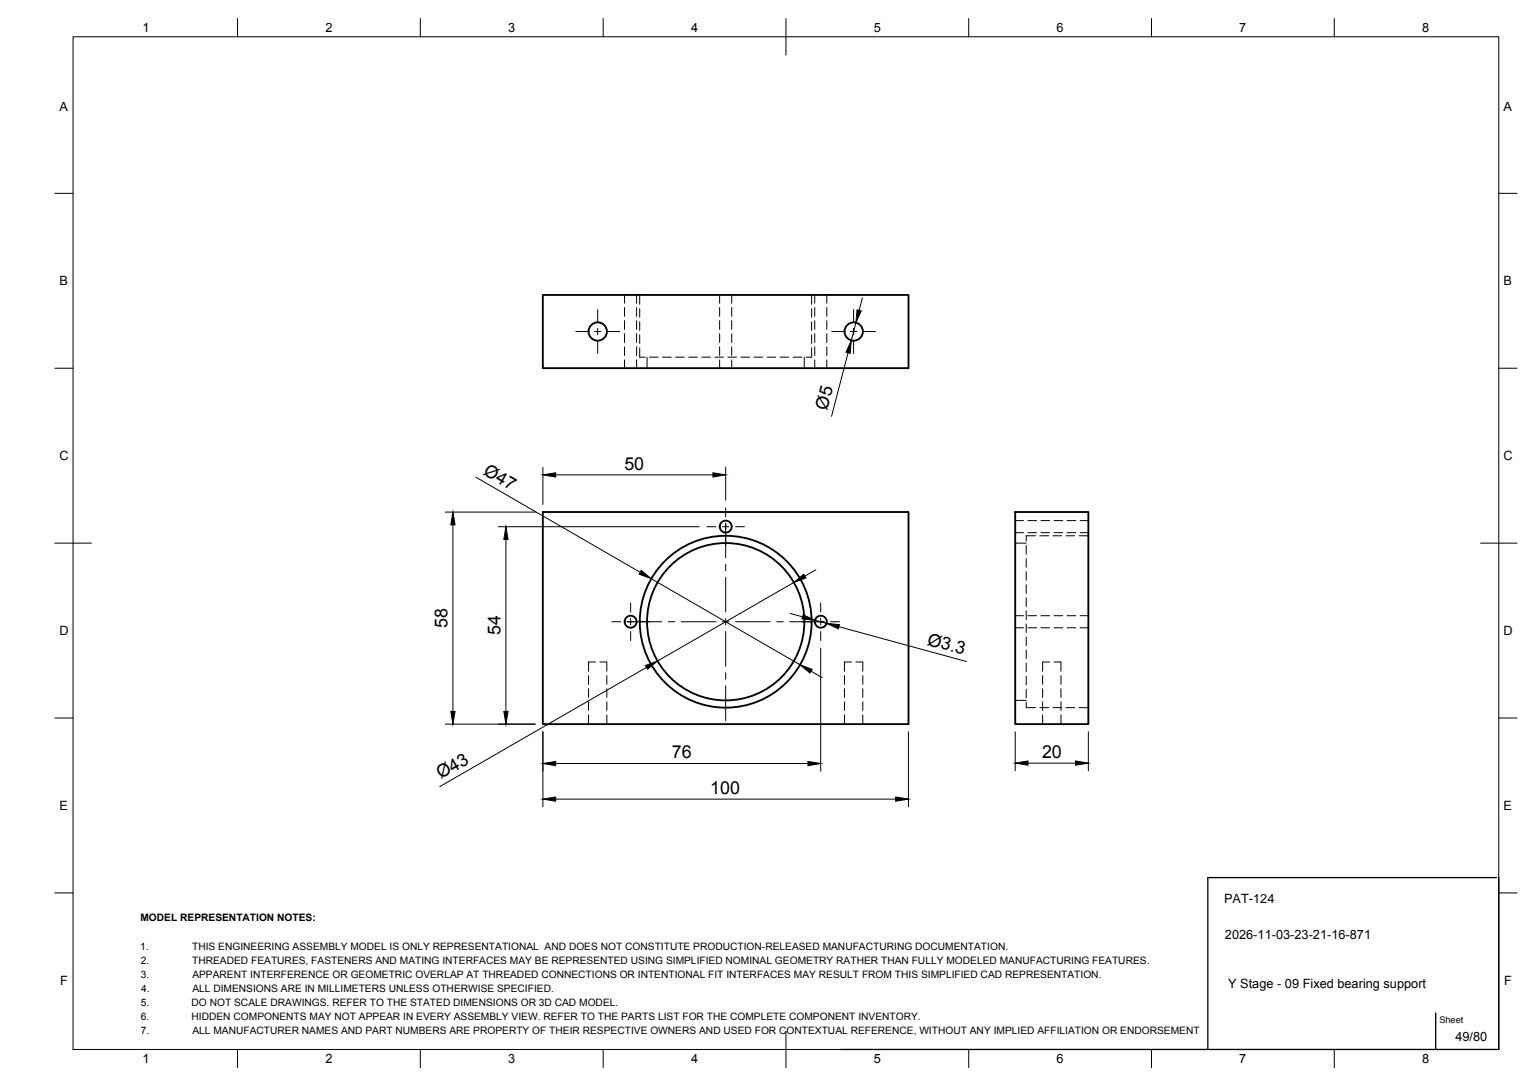
ISO-10303-21;
HEADER;
/* Generated by software containing ST-Developer
 * from STEP Tools, Inc. (www.steptools.com) 
 */

FILE_DESCRIPTION(
/* description */ ('XY cross-slide table'),
/* implementation_level */ '2;1');

FILE_NAME(
/* name */ 'Y Stage - 09 Fixed bearing support.step',
/* time_stamp */ '2026-10-28T03:22:46-07:00',
/* author */ (''),
/* organization */ (''),
/* preprocessor_version */ 'ST-DEVELOPER v20.2',
/* originating_system */ 'Autodesk Translation Framework v15.17.0.0',
/* authorisation */ '');

FILE_SCHEMA (('AUTOMOTIVE_DESIGN { 1 0 10303 214 3 1 1 }'));
ENDSEC;

DATA;
#10=MECHANICAL_DESIGN_GEOMETRIC_PRESENTATION_REPRESENTATION('',(#1731),#62984);
#1550=SHAPE_REPRESENTATION_RELATIONSHIP('SRR','None',#63405,#1633);
#1633=ADVANCED_BREP_SHAPE_REPRESENTATION('',(#1840),#62942);
#1731=STYLED_ITEM('',(#63912),#1840);
#1840=MANIFOLD_SOLID_BREP('Body1',#23029);
#2163=FACE_BOUND('',#5200,.T.);
#2164=FACE_BOUND('',#5208,.T.);
#2165=FACE_BOUND('',#5209,.T.);
#2166=FACE_BOUND('',#5210,.T.);
#2167=FACE_BOUND('',#5211,.T.);
#2168=FACE_BOUND('',#5214,.T.);
#2169=FACE_BOUND('',#5215,.T.);
#2170=FACE_BOUND('',#5216,.T.);
#2171=FACE_BOUND('',#5217,.T.);
#2172=FACE_BOUND('',#5220,.T.);
#2173=FACE_BOUND('',#5221,.T.);
#2617=PLANE('',#25418);
#2618=PLANE('',#25425);
#2619=PLANE('',#25429);
#2620=PLANE('',#25430);
#2621=PLANE('',#25431);
#2622=PLANE('',#25432);
#2623=PLANE('',#25433);
#2624=PLANE('',#25434);
#2625=PLANE('',#25435);
#3605=FACE_OUTER_BOUND('',#5195,.T.);
#3606=FACE_OUTER_BOUND('',#5196,.T.);
#3607=FACE_OUTER_BOUND('',#5197,.T.);
#3608=FACE_OUTER_BOUND('',#5198,.T.);
#3609=FACE_OUTER_BOUND('',#5199,.T.);
#3610=FACE_OUTER_BOUND('',#5201,.T.);
#3611=FACE_OUTER_BOUND('',#5202,.T.);
#3612=FACE_OUTER_BOUND('',#5203,.T.);
#3613=FACE_OUTER_BOUND('',#5204,.T.);
#3614=FACE_OUTER_BOUND('',#5205,.T.);
#3615=FACE_OUTER_BOUND('',#5206,.T.);
#3616=FACE_OUTER_BOUND('',#5207,.T.);
#3617=FACE_OUTER_BOUND('',#5212,.T.);
#3618=FACE_OUTER_BOUND('',#5213,.T.);
#3619=FACE_OUTER_BOUND('',#5218,.T.);
#3620=FACE_OUTER_BOUND('',#5219,.T.);
#5195=EDGE_LOOP('',(#18328,#18329,#18330,#18331));
#5196=EDGE_LOOP('',(#18332,#18333,#18334,#18335));
#5197=EDGE_LOOP('',(#18336,#18337,#18338,#18339));
#5198=EDGE_LOOP('',(#18340,#18341,#18342,#18343));
#5199=EDGE_LOOP('',(#18344));
#5200=EDGE_LOOP('',(#18345));
#5201=EDGE_LOOP('',(#18346,#18347,#18348,#18349));
#5202=EDGE_LOOP('',(#18350,#18351,#18352,#18353));
#5203=EDGE_LOOP('',(#18354));
#5204=EDGE_LOOP('',(#18355,#18356,#18357,#18358));
#5205=EDGE_LOOP('',(#18359));
#5206=EDGE_LOOP('',(#18360,#18361,#18362,#18363));
#5207=EDGE_LOOP('',(#18364,#18365,#18366,#18367));
#5208=EDGE_LOOP('',(#18368));
#5209=EDGE_LOOP('',(#18369));
#5210=EDGE_LOOP('',(#18370));
#5211=EDGE_LOOP('',(#18371));
#5212=EDGE_LOOP('',(#18372,#18373,#18374,#18375));
#5213=EDGE_LOOP('',(#18376,#18377,#18378,#18379));
#5214=EDGE_LOOP('',(#18380));
#5215=EDGE_LOOP('',(#18381));
#5216=EDGE_LOOP('',(#18382));
#5217=EDGE_LOOP('',(#18383));
#5218=EDGE_LOOP('',(#18384,#18385,#18386,#18387));
#5219=EDGE_LOOP('',(#18388,#18389,#18390,#18391));
#5220=EDGE_LOOP('',(#18392));
#5221=EDGE_LOOP('',(#18393));
#6737=LINE('',#48212,#8224);
#6738=LINE('',#48218,#8225);
#6739=LINE('',#48224,#8226);
#6740=LINE('',#48230,#8227);
#6741=LINE('',#48238,#8228);
#6742=LINE('',#48243,#8229);
#6743=LINE('',#48250,#8230);
#6744=LINE('',#48256,#8231);
#6745=LINE('',#48258,#8232);
#6746=LINE('',#48260,#8233);
#6747=LINE('',#48261,#8234);
#6748=LINE('',#48264,#8235);
#6749=LINE('',#48266,#8236);
#6750=LINE('',#48267,#8237);
#6751=LINE('',#48270,#8238);
#6752=LINE('',#48272,#8239);
#6753=LINE('',#48273,#8240);
#6754=LINE('',#48275,#8241);
#6755=LINE('',#48276,#8242);
#8224=VECTOR('',#30108,0.165);
#8225=VECTOR('',#30115,0.165);
#8226=VECTOR('',#30122,0.165);
#8227=VECTOR('',#30129,2.35);
#8228=VECTOR('',#30140,2.15);
#8229=VECTOR('',#30145,0.25);
#8230=VECTOR('',#30154,0.25);
#8231=VECTOR('',#30161,1.);
#8232=VECTOR('',#30162,1.);
#8233=VECTOR('',#30163,1.);
#8234=VECTOR('',#30164,1.);
#8235=VECTOR('',#30167,1.);
#8236=VECTOR('',#30168,1.);
#8237=VECTOR('',#30169,1.);
#8238=VECTOR('',#30172,1.);
#8239=VECTOR('',#30173,1.);
#8240=VECTOR('',#30174,1.);
#8241=VECTOR('',#30177,1.);
#8242=VECTOR('',#30178,1.);
#9417=CIRCLE('',#25407,0.165);
#9418=CIRCLE('',#25408,0.165);
#9419=CIRCLE('',#25410,0.165);
#9420=CIRCLE('',#25411,0.165);
#9421=CIRCLE('',#25413,0.165);
#9422=CIRCLE('',#25414,0.165);
#9423=CIRCLE('',#25416,2.35);
#9424=CIRCLE('',#25417,2.35);
#9425=CIRCLE('',#25419,2.15);
#9426=CIRCLE('',#25421,2.15);
#9427=CIRCLE('',#25423,0.25);
#9428=CIRCLE('',#25424,0.25);
#9429=CIRCLE('',#25427,0.25);
#9430=CIRCLE('',#25428,0.25);
#10921=VERTEX_POINT('',#48209);
#10922=VERTEX_POINT('',#48211);
#10923=VERTEX_POINT('',#48215);
#10924=VERTEX_POINT('',#48217);
#10925=VERTEX_POINT('',#48221);
#10926=VERTEX_POINT('',#48223);
#10927=VERTEX_POINT('',#48227);
#10928=VERTEX_POINT('',#48229);
#10929=VERTEX_POINT('',#48233);
#10930=VERTEX_POINT('',#48236);
#10931=VERTEX_POINT('',#48240);
#10932=VERTEX_POINT('',#48242);
#10933=VERTEX_POINT('',#48247);
#10934=VERTEX_POINT('',#48249);
#10935=VERTEX_POINT('',#48254);
#10936=VERTEX_POINT('',#48255);
#10937=VERTEX_POINT('',#48257);
#10938=VERTEX_POINT('',#48259);
#10939=VERTEX_POINT('',#48263);
#10940=VERTEX_POINT('',#48265);
#10941=VERTEX_POINT('',#48269);
#10942=VERTEX_POINT('',#48271);
#13548=EDGE_CURVE('',#10921,#10921,#9417,.T.);
#13549=EDGE_CURVE('',#10921,#10922,#6737,.T.);
#13550=EDGE_CURVE('',#10922,#10922,#9418,.T.);
#13551=EDGE_CURVE('',#10923,#10923,#9419,.T.);
#13552=EDGE_CURVE('',#10923,#10924,#6738,.T.);
#13553=EDGE_CURVE('',#10924,#10924,#9420,.T.);
#13554=EDGE_CURVE('',#10925,#10925,#9421,.T.);
#13555=EDGE_CURVE('',#10925,#10926,#6739,.T.);
#13556=EDGE_CURVE('',#10926,#10926,#9422,.T.);
#13557=EDGE_CURVE('',#10927,#10927,#9423,.T.);
#13558=EDGE_CURVE('',#10927,#10928,#6740,.T.);
#13559=EDGE_CURVE('',#10928,#10928,#9424,.T.);
#13560=EDGE_CURVE('',#10929,#10929,#9425,.T.);
#13561=EDGE_CURVE('',#10930,#10930,#9426,.T.);
#13562=EDGE_CURVE('',#10930,#10929,#6741,.T.);
#13563=EDGE_CURVE('',#10931,#10931,#9427,.T.);
#13564=EDGE_CURVE('',#10931,#10932,#6742,.T.);
#13565=EDGE_CURVE('',#10932,#10932,#9428,.T.);
#13566=EDGE_CURVE('',#10933,#10933,#9429,.T.);
#13567=EDGE_CURVE('',#10933,#10934,#6743,.T.);
#13568=EDGE_CURVE('',#10934,#10934,#9430,.T.);
#13569=EDGE_CURVE('',#10935,#10936,#6744,.T.);
#13570=EDGE_CURVE('',#10936,#10937,#6745,.T.);
#13571=EDGE_CURVE('',#10938,#10937,#6746,.T.);
#13572=EDGE_CURVE('',#10935,#10938,#6747,.T.);
#13573=EDGE_CURVE('',#10939,#10935,#6748,.T.);
#13574=EDGE_CURVE('',#10940,#10938,#6749,.T.);
#13575=EDGE_CURVE('',#10939,#10940,#6750,.T.);
#13576=EDGE_CURVE('',#10941,#10939,#6751,.T.);
#13577=EDGE_CURVE('',#10942,#10940,#6752,.T.);
#13578=EDGE_CURVE('',#10941,#10942,#6753,.T.);
#13579=EDGE_CURVE('',#10936,#10941,#6754,.T.);
#13580=EDGE_CURVE('',#10937,#10942,#6755,.T.);
#18328=ORIENTED_EDGE('',*,*,#13548,.F.);
#18329=ORIENTED_EDGE('',*,*,#13549,.T.);
#18330=ORIENTED_EDGE('',*,*,#13550,.F.);
#18331=ORIENTED_EDGE('',*,*,#13549,.F.);
#18332=ORIENTED_EDGE('',*,*,#13551,.F.);
#18333=ORIENTED_EDGE('',*,*,#13552,.T.);
#18334=ORIENTED_EDGE('',*,*,#13553,.F.);
#18335=ORIENTED_EDGE('',*,*,#13552,.F.);
#18336=ORIENTED_EDGE('',*,*,#13554,.F.);
#18337=ORIENTED_EDGE('',*,*,#13555,.T.);
#18338=ORIENTED_EDGE('',*,*,#13556,.F.);
#18339=ORIENTED_EDGE('',*,*,#13555,.F.);
#18340=ORIENTED_EDGE('',*,*,#13557,.F.);
#18341=ORIENTED_EDGE('',*,*,#13558,.T.);
#18342=ORIENTED_EDGE('',*,*,#13559,.F.);
#18343=ORIENTED_EDGE('',*,*,#13558,.F.);
#18344=ORIENTED_EDGE('',*,*,#13557,.T.);
#18345=ORIENTED_EDGE('',*,*,#13560,.F.);
#18346=ORIENTED_EDGE('',*,*,#13561,.F.);
#18347=ORIENTED_EDGE('',*,*,#13562,.T.);
#18348=ORIENTED_EDGE('',*,*,#13560,.T.);
#18349=ORIENTED_EDGE('',*,*,#13562,.F.);
#18350=ORIENTED_EDGE('',*,*,#13563,.F.);
#18351=ORIENTED_EDGE('',*,*,#13564,.T.);
#18352=ORIENTED_EDGE('',*,*,#13565,.T.);
#18353=ORIENTED_EDGE('',*,*,#13564,.F.);
#18354=ORIENTED_EDGE('',*,*,#13565,.F.);
#18355=ORIENTED_EDGE('',*,*,#13566,.F.);
#18356=ORIENTED_EDGE('',*,*,#13567,.T.);
#18357=ORIENTED_EDGE('',*,*,#13568,.T.);
#18358=ORIENTED_EDGE('',*,*,#13567,.F.);
#18359=ORIENTED_EDGE('',*,*,#13568,.F.);
#18360=ORIENTED_EDGE('',*,*,#13569,.T.);
#18361=ORIENTED_EDGE('',*,*,#13570,.T.);
#18362=ORIENTED_EDGE('',*,*,#13571,.F.);
#18363=ORIENTED_EDGE('',*,*,#13572,.F.);
#18364=ORIENTED_EDGE('',*,*,#13573,.T.);
#18365=ORIENTED_EDGE('',*,*,#13572,.T.);
#18366=ORIENTED_EDGE('',*,*,#13574,.F.);
#18367=ORIENTED_EDGE('',*,*,#13575,.F.);
#18368=ORIENTED_EDGE('',*,*,#13550,.T.);
#18369=ORIENTED_EDGE('',*,*,#13553,.T.);
#18370=ORIENTED_EDGE('',*,*,#13556,.T.);
#18371=ORIENTED_EDGE('',*,*,#13559,.T.);
#18372=ORIENTED_EDGE('',*,*,#13576,.T.);
#18373=ORIENTED_EDGE('',*,*,#13575,.T.);
#18374=ORIENTED_EDGE('',*,*,#13577,.F.);
#18375=ORIENTED_EDGE('',*,*,#13578,.F.);
#18376=ORIENTED_EDGE('',*,*,#13579,.T.);
#18377=ORIENTED_EDGE('',*,*,#13578,.T.);
#18378=ORIENTED_EDGE('',*,*,#13580,.F.);
#18379=ORIENTED_EDGE('',*,*,#13570,.F.);
#18380=ORIENTED_EDGE('',*,*,#13548,.T.);
#18381=ORIENTED_EDGE('',*,*,#13551,.T.);
#18382=ORIENTED_EDGE('',*,*,#13554,.T.);
#18383=ORIENTED_EDGE('',*,*,#13561,.T.);
#18384=ORIENTED_EDGE('',*,*,#13580,.T.);
#18385=ORIENTED_EDGE('',*,*,#13577,.T.);
#18386=ORIENTED_EDGE('',*,*,#13574,.T.);
#18387=ORIENTED_EDGE('',*,*,#13571,.T.);
#18388=ORIENTED_EDGE('',*,*,#13579,.F.);
#18389=ORIENTED_EDGE('',*,*,#13569,.F.);
#18390=ORIENTED_EDGE('',*,*,#13573,.F.);
#18391=ORIENTED_EDGE('',*,*,#13576,.F.);
#18392=ORIENTED_EDGE('',*,*,#13563,.T.);
#18393=ORIENTED_EDGE('',*,*,#13566,.T.);
#21391=CYLINDRICAL_SURFACE('',#25406,0.165);
#21392=CYLINDRICAL_SURFACE('',#25409,0.165);
#21393=CYLINDRICAL_SURFACE('',#25412,0.165);
#21394=CYLINDRICAL_SURFACE('',#25415,2.35);
#21395=CYLINDRICAL_SURFACE('',#25420,2.15);
#21396=CYLINDRICAL_SURFACE('',#25422,0.25);
#21397=CYLINDRICAL_SURFACE('',#25426,0.25);
#22386=ADVANCED_FACE('',(#3605),#21391,.F.);
#22387=ADVANCED_FACE('',(#3606),#21392,.F.);
#22388=ADVANCED_FACE('',(#3607),#21393,.F.);
#22389=ADVANCED_FACE('',(#3608),#21394,.F.);
#22390=ADVANCED_FACE('',(#3609,#2163),#2617,.T.);
#22391=ADVANCED_FACE('',(#3610),#21395,.F.);
#22392=ADVANCED_FACE('',(#3611),#21396,.F.);
#22393=ADVANCED_FACE('',(#3612),#2618,.F.);
#22394=ADVANCED_FACE('',(#3613),#21397,.F.);
#22395=ADVANCED_FACE('',(#3614),#2619,.F.);
#22396=ADVANCED_FACE('',(#3615),#2620,.T.);
#22397=ADVANCED_FACE('',(#3616,#2164,#2165,#2166,#2167),#2621,.T.);
#22398=ADVANCED_FACE('',(#3617),#2622,.T.);
#22399=ADVANCED_FACE('',(#3618,#2168,#2169,#2170,#2171),#2623,.T.);
#22400=ADVANCED_FACE('',(#3619),#2624,.T.);
#22401=ADVANCED_FACE('',(#3620,#2172,#2173),#2625,.F.);
#23029=CLOSED_SHELL('',(#22386,#22387,#22388,#22389,#22390,#22391,#22392,
#22393,#22394,#22395,#22396,#22397,#22398,#22399,#22400,#22401));
#25405=AXIS2_PLACEMENT_3D('',#48207,#30102,#30103);
#25406=AXIS2_PLACEMENT_3D('',#48208,#30104,#30105);
#25407=AXIS2_PLACEMENT_3D('',#48210,#30106,#30107);
#25408=AXIS2_PLACEMENT_3D('',#48213,#30109,#30110);
#25409=AXIS2_PLACEMENT_3D('',#48214,#30111,#30112);
#25410=AXIS2_PLACEMENT_3D('',#48216,#30113,#30114);
#25411=AXIS2_PLACEMENT_3D('',#48219,#30116,#30117);
#25412=AXIS2_PLACEMENT_3D('',#48220,#30118,#30119);
#25413=AXIS2_PLACEMENT_3D('',#48222,#30120,#30121);
#25414=AXIS2_PLACEMENT_3D('',#48225,#30123,#30124);
#25415=AXIS2_PLACEMENT_3D('',#48226,#30125,#30126);
#25416=AXIS2_PLACEMENT_3D('',#48228,#30127,#30128);
#25417=AXIS2_PLACEMENT_3D('',#48231,#30130,#30131);
#25418=AXIS2_PLACEMENT_3D('',#48232,#30132,#30133);
#25419=AXIS2_PLACEMENT_3D('',#48234,#30134,#30135);
#25420=AXIS2_PLACEMENT_3D('',#48235,#30136,#30137);
#25421=AXIS2_PLACEMENT_3D('',#48237,#30138,#30139);
#25422=AXIS2_PLACEMENT_3D('',#48239,#30141,#30142);
#25423=AXIS2_PLACEMENT_3D('',#48241,#30143,#30144);
#25424=AXIS2_PLACEMENT_3D('',#48244,#30146,#30147);
#25425=AXIS2_PLACEMENT_3D('',#48245,#30148,#30149);
#25426=AXIS2_PLACEMENT_3D('',#48246,#30150,#30151);
#25427=AXIS2_PLACEMENT_3D('',#48248,#30152,#30153);
#25428=AXIS2_PLACEMENT_3D('',#48251,#30155,#30156);
#25429=AXIS2_PLACEMENT_3D('',#48252,#30157,#30158);
#25430=AXIS2_PLACEMENT_3D('',#48253,#30159,#30160);
#25431=AXIS2_PLACEMENT_3D('',#48262,#30165,#30166);
#25432=AXIS2_PLACEMENT_3D('',#48268,#30170,#30171);
#25433=AXIS2_PLACEMENT_3D('',#48274,#30175,#30176);
#25434=AXIS2_PLACEMENT_3D('',#48277,#30179,#30180);
#25435=AXIS2_PLACEMENT_3D('',#48278,#30181,#30182);
#30102=DIRECTION('axis',(0.,0.,1.));
#30103=DIRECTION('refdir',(1.,0.,0.));
#30104=DIRECTION('center_axis',(1.,0.,0.));
#30105=DIRECTION('ref_axis',(0.,0.,-1.));
#30106=DIRECTION('center_axis',(1.,0.,0.));
#30107=DIRECTION('ref_axis',(0.,0.,-1.));
#30108=DIRECTION('',(1.,0.,0.));
#30109=DIRECTION('center_axis',(-1.,0.,0.));
#30110=DIRECTION('ref_axis',(0.,0.,-1.));
#30111=DIRECTION('center_axis',(1.,0.,0.));
#30112=DIRECTION('ref_axis',(0.,0.,-1.));
#30113=DIRECTION('center_axis',(1.,0.,0.));
#30114=DIRECTION('ref_axis',(0.,0.,-1.));
#30115=DIRECTION('',(1.,0.,0.));
#30116=DIRECTION('center_axis',(-1.,0.,0.));
#30117=DIRECTION('ref_axis',(0.,0.,-1.));
#30118=DIRECTION('center_axis',(1.,0.,0.));
#30119=DIRECTION('ref_axis',(0.,0.,-1.));
#30120=DIRECTION('center_axis',(1.,0.,0.));
#30121=DIRECTION('ref_axis',(0.,0.,-1.));
#30122=DIRECTION('',(1.,0.,0.));
#30123=DIRECTION('center_axis',(-1.,0.,0.));
#30124=DIRECTION('ref_axis',(0.,0.,-1.));
#30125=DIRECTION('center_axis',(1.,0.,0.));
#30126=DIRECTION('ref_axis',(0.,0.,-1.));
#30127=DIRECTION('center_axis',(1.,0.,0.));
#30128=DIRECTION('ref_axis',(0.,0.,-1.));
#30129=DIRECTION('',(1.,0.,0.));
#30130=DIRECTION('center_axis',(-1.,0.,0.));
#30131=DIRECTION('ref_axis',(0.,0.,-1.));
#30132=DIRECTION('center_axis',(1.,0.,0.));
#30133=DIRECTION('ref_axis',(0.,0.,-1.));
#30134=DIRECTION('center_axis',(1.,0.,0.));
#30135=DIRECTION('ref_axis',(0.,0.,-1.));
#30136=DIRECTION('center_axis',(1.,0.,0.));
#30137=DIRECTION('ref_axis',(0.,0.,-1.));
#30138=DIRECTION('center_axis',(1.,0.,0.));
#30139=DIRECTION('ref_axis',(0.,0.,-1.));
#30140=DIRECTION('',(1.,0.,0.));
#30141=DIRECTION('center_axis',(0.,0.,1.));
#30142=DIRECTION('ref_axis',(1.,0.,0.));
#30143=DIRECTION('center_axis',(0.,0.,1.));
#30144=DIRECTION('ref_axis',(1.,0.,0.));
#30145=DIRECTION('',(0.,0.,1.));
#30146=DIRECTION('center_axis',(0.,0.,1.));
#30147=DIRECTION('ref_axis',(1.,0.,0.));
#30148=DIRECTION('center_axis',(0.,0.,1.));
#30149=DIRECTION('ref_axis',(1.,0.,0.));
#30150=DIRECTION('center_axis',(0.,0.,1.));
#30151=DIRECTION('ref_axis',(1.,0.,0.));
#30152=DIRECTION('center_axis',(0.,0.,1.));
#30153=DIRECTION('ref_axis',(1.,0.,0.));
#30154=DIRECTION('',(0.,0.,1.));
#30155=DIRECTION('center_axis',(0.,0.,1.));
#30156=DIRECTION('ref_axis',(1.,0.,0.));
#30157=DIRECTION('center_axis',(0.,0.,1.));
#30158=DIRECTION('ref_axis',(1.,0.,0.));
#30159=DIRECTION('center_axis',(0.,1.,0.));
#30160=DIRECTION('ref_axis',(-1.,0.,0.));
#30161=DIRECTION('',(-1.,0.,0.));
#30162=DIRECTION('',(0.,0.,1.));
#30163=DIRECTION('',(-1.,0.,0.));
#30164=DIRECTION('',(0.,0.,1.));
#30165=DIRECTION('center_axis',(1.,0.,0.));
#30166=DIRECTION('ref_axis',(0.,1.,0.));
#30167=DIRECTION('',(0.,1.,0.));
#30168=DIRECTION('',(0.,1.,0.));
#30169=DIRECTION('',(0.,0.,1.));
#30170=DIRECTION('center_axis',(0.,-1.,0.));
#30171=DIRECTION('ref_axis',(1.,0.,0.));
#30172=DIRECTION('',(1.,0.,0.));
#30173=DIRECTION('',(1.,0.,0.));
#30174=DIRECTION('',(0.,0.,1.));
#30175=DIRECTION('center_axis',(-1.,0.,0.));
#30176=DIRECTION('ref_axis',(0.,-1.,0.));
#30177=DIRECTION('',(0.,-1.,0.));
#30178=DIRECTION('',(0.,-1.,0.));
#30179=DIRECTION('center_axis',(0.,0.,1.));
#30180=DIRECTION('ref_axis',(1.,0.,0.));
#30181=DIRECTION('center_axis',(0.,0.,1.));
#30182=DIRECTION('ref_axis',(1.,0.,0.));
#48207=CARTESIAN_POINT('',(0.,0.,0.));
#48208=CARTESIAN_POINT('Origin',(22.9,-2.6,4.));
#48209=CARTESIAN_POINT('',(23.,-2.6,4.165));
#48210=CARTESIAN_POINT('Origin',(23.,-2.6,4.));
#48211=CARTESIAN_POINT('',(25.,-2.6,4.165));
#48212=CARTESIAN_POINT('',(22.9,-2.6,4.165));
#48213=CARTESIAN_POINT('Origin',(25.,-2.6,4.));
#48214=CARTESIAN_POINT('Origin',(22.9,2.6,4.));
#48215=CARTESIAN_POINT('',(23.,2.6,4.165));
#48216=CARTESIAN_POINT('Origin',(23.,2.6,4.));
#48217=CARTESIAN_POINT('',(25.,2.6,4.165));
#48218=CARTESIAN_POINT('',(22.9,2.6,4.165));
#48219=CARTESIAN_POINT('Origin',(25.,2.6,4.));
#48220=CARTESIAN_POINT('Origin',(22.9,0.,6.6));
#48221=CARTESIAN_POINT('',(23.,-2.02066721859313E-17,6.765));
#48222=CARTESIAN_POINT('Origin',(23.,0.,6.6));
#48223=CARTESIAN_POINT('',(25.,2.02066721859313E-17,6.765));
#48224=CARTESIAN_POINT('',(22.9,-2.02066721859313E-17,6.765));
#48225=CARTESIAN_POINT('Origin',(25.,0.,6.6));
#48226=CARTESIAN_POINT('Origin',(23.3,0.,4.));
#48227=CARTESIAN_POINT('',(23.3,-2.87791997799628E-16,6.35));
#48228=CARTESIAN_POINT('Origin',(23.3,0.,4.));
#48229=CARTESIAN_POINT('',(25.,2.87791997799628E-16,6.35));
#48230=CARTESIAN_POINT('',(23.3,-2.87791997799628E-16,6.35));
#48231=CARTESIAN_POINT('Origin',(25.,0.,4.));
#48232=CARTESIAN_POINT('Origin',(23.3,0.,4.));
#48233=CARTESIAN_POINT('',(23.3,-2.63299061816681E-16,6.15));
#48234=CARTESIAN_POINT('Origin',(23.3,0.,4.));
#48235=CARTESIAN_POINT('Origin',(22.9,0.,4.));
#48236=CARTESIAN_POINT('',(23.,-2.63299061816681E-16,6.15));
#48237=CARTESIAN_POINT('Origin',(23.,0.,4.));
#48238=CARTESIAN_POINT('',(22.9,-2.63299061816681E-16,6.15));
#48239=CARTESIAN_POINT('Origin',(24.,-3.5,1.1));
#48240=CARTESIAN_POINT('',(23.75,-3.5,1.2));
#48241=CARTESIAN_POINT('Origin',(24.,-3.5,1.2));
#48242=CARTESIAN_POINT('',(23.75,-3.5,2.9));
#48243=CARTESIAN_POINT('',(23.75,-3.5,1.1));
#48244=CARTESIAN_POINT('Origin',(24.,-3.5,2.9));
#48245=CARTESIAN_POINT('Origin',(24.,-3.5,2.9));
#48246=CARTESIAN_POINT('Origin',(24.,3.5,1.1));
#48247=CARTESIAN_POINT('',(23.75,3.5,1.2));
#48248=CARTESIAN_POINT('Origin',(24.,3.5,1.2));
#48249=CARTESIAN_POINT('',(23.75,3.5,2.9));
#48250=CARTESIAN_POINT('',(23.75,3.5,1.1));
#48251=CARTESIAN_POINT('Origin',(24.,3.5,2.9));
#48252=CARTESIAN_POINT('Origin',(24.,3.5,2.9));
#48253=CARTESIAN_POINT('Origin',(25.,5.,1.2));
#48254=CARTESIAN_POINT('',(25.,5.,1.2));
#48255=CARTESIAN_POINT('',(23.,5.,1.2));
#48256=CARTESIAN_POINT('',(25.,5.,1.2));
#48257=CARTESIAN_POINT('',(23.,5.,7.));
#48258=CARTESIAN_POINT('',(23.,5.,1.2));
#48259=CARTESIAN_POINT('',(25.,5.,7.));
#48260=CARTESIAN_POINT('',(25.,5.,7.));
#48261=CARTESIAN_POINT('',(25.,5.,1.2));
#48262=CARTESIAN_POINT('Origin',(25.,-5.,1.2));
#48263=CARTESIAN_POINT('',(25.,-5.,1.2));
#48264=CARTESIAN_POINT('',(25.,-5.,1.2));
#48265=CARTESIAN_POINT('',(25.,-5.,7.));
#48266=CARTESIAN_POINT('',(25.,-5.,7.));
#48267=CARTESIAN_POINT('',(25.,-5.,1.2));
#48268=CARTESIAN_POINT('Origin',(23.,-5.,1.2));
#48269=CARTESIAN_POINT('',(23.,-5.,1.2));
#48270=CARTESIAN_POINT('',(23.,-5.,1.2));
#48271=CARTESIAN_POINT('',(23.,-5.,7.));
#48272=CARTESIAN_POINT('',(23.,-5.,7.));
#48273=CARTESIAN_POINT('',(23.,-5.,1.2));
#48274=CARTESIAN_POINT('Origin',(23.,5.,1.2));
#48275=CARTESIAN_POINT('',(23.,5.,1.2));
#48276=CARTESIAN_POINT('',(23.,5.,7.));
#48277=CARTESIAN_POINT('Origin',(24.,0.,7.));
#48278=CARTESIAN_POINT('Origin',(24.,0.,1.2));
#62843=UNCERTAINTY_MEASURE_WITH_UNIT(LENGTH_MEASURE(0.001),#62985,
'DISTANCE_ACCURACY_VALUE',
'Maximum model space distance between geometric entities at asserted c
onnectivities');
#62885=UNCERTAINTY_MEASURE_WITH_UNIT(LENGTH_MEASURE(0.001),#62985,
'DISTANCE_ACCURACY_VALUE',
'Maximum model space distance between geometric entities at asserted c
onnectivities');
#62942=(
GEOMETRIC_REPRESENTATION_CONTEXT(3)
GLOBAL_UNCERTAINTY_ASSIGNED_CONTEXT((#62843))
GLOBAL_UNIT_ASSIGNED_CONTEXT((#62985,#62987,#62988))
REPRESENTATION_CONTEXT('','3D')
);
#62984=(
GEOMETRIC_REPRESENTATION_CONTEXT(3)
GLOBAL_UNCERTAINTY_ASSIGNED_CONTEXT((#62885))
GLOBAL_UNIT_ASSIGNED_CONTEXT((#62985,#62987,#62988))
REPRESENTATION_CONTEXT('','3D')
);
#62985=(
LENGTH_UNIT()
NAMED_UNIT(*)
SI_UNIT(.CENTI.,.METRE.)
);
#62987=(
NAMED_UNIT(*)
PLANE_ANGLE_UNIT()
SI_UNIT($,.RADIAN.)
);
#62988=(
NAMED_UNIT(*)
SI_UNIT($,.STERADIAN.)
SOLID_ANGLE_UNIT()
);
#63045=SHAPE_DEFINITION_REPRESENTATION(#63223,#63405);
#63223=PRODUCT_DEFINITION_SHAPE('',$,#63504);
#63405=SHAPE_REPRESENTATION('',(#25405),#62942);
#63447=PRODUCT_DEFINITION_CONTEXT('part definition',#63743,'design');
#63504=PRODUCT_DEFINITION('Y Stage - 09 Fixed bearing support',
'Y Stage - 09 Fixed bearing support',#63602,#63447);
#63602=PRODUCT_DEFINITION_FORMATION('',$,#63801);
#63743=APPLICATION_CONTEXT(
'Core Data for Automotive Mechanical Design Process');
#63744=PRODUCT_CONTEXT('part definition',#63743,'mechanical');
#63801=PRODUCT('Y Stage - 09 Fixed bearing support',
'Y Stage - 09 Fixed bearing support',
'Y Stage - 09 Fixed bearing support',(#63744));
#63906=COLOUR_RGB('Grey',0.48,0.52,0.57);
#63907=FILL_AREA_STYLE_COLOUR('',#63906);
#63908=FILL_AREA_STYLE('',(#63907));
#63909=SURFACE_STYLE_FILL_AREA(#63908);
#63910=SURFACE_SIDE_STYLE('',(#63909));
#63911=SURFACE_STYLE_USAGE(.BOTH.,#63910);
#63912=PRESENTATION_STYLE_ASSIGNMENT((#63911));
ENDSEC;
END-ISO-10303-21;
